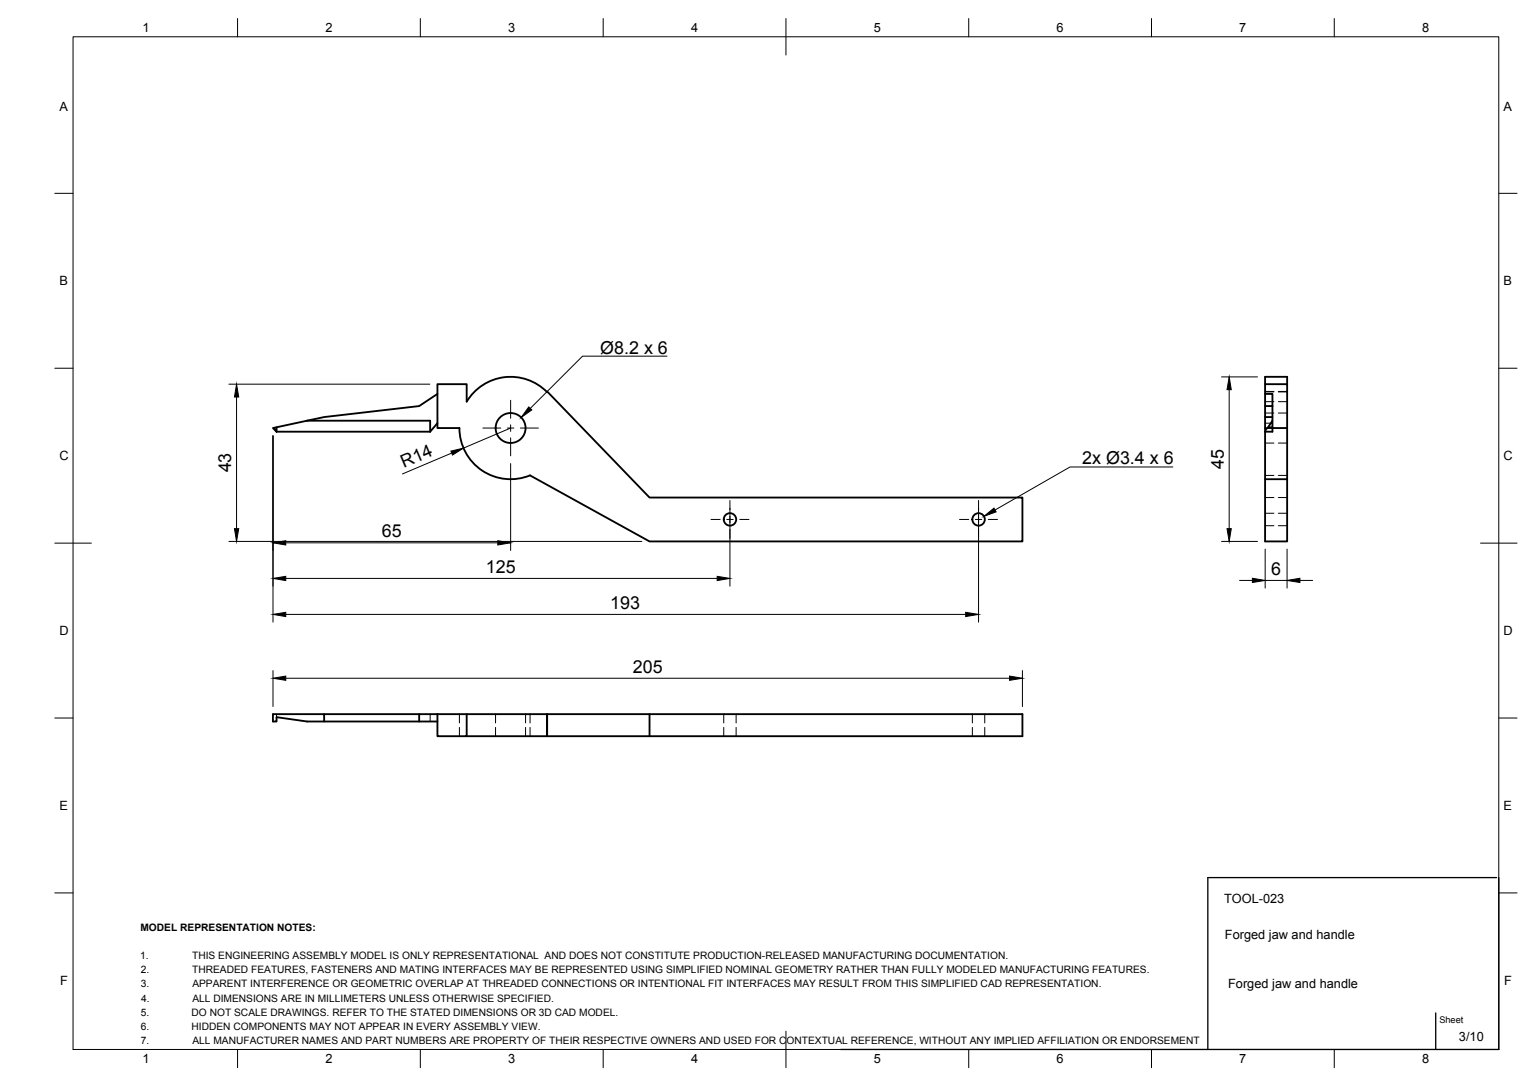
ISO-10303-21;
HEADER;
/* Generated by software containing ST-Developer
 * from STEP Tools, Inc. (www.steptools.com) 
 */

FILE_DESCRIPTION(
/* description */ (''),
/* implementation_level */ '2;1');

FILE_NAME(
/* name */ 'Forged jaw and handle.step',
/* time_stamp */ '2026-11-10T05:40:20-08:00',
/* author */ (''),
/* organization */ (''),
/* preprocessor_version */ 'ST-DEVELOPER v20.2',
/* originating_system */ 'Autodesk Translation Framework v15.17.0.0',
/* authorisation */ '');

FILE_SCHEMA (('AUTOMOTIVE_DESIGN { 1 0 10303 214 3 1 1 }'));
ENDSEC;

DATA;
#10=MECHANICAL_DESIGN_GEOMETRIC_PRESENTATION_REPRESENTATION('',(#572),#18580);
#554=SHAPE_REPRESENTATION_RELATIONSHIP('SRR','None',#18624,#563);
#563=ADVANCED_BREP_SHAPE_REPRESENTATION('',(#581),#18570);
#572=STYLED_ITEM('',(#18683),#581);
#581=MANIFOLD_SOLID_BREP('Body1',#6544);
#590=FACE_BOUND('',#1186,.T.);
#591=FACE_BOUND('',#1187,.T.);
#592=FACE_BOUND('',#1188,.T.);
#593=FACE_BOUND('',#1196,.T.);
#594=FACE_BOUND('',#1197,.T.);
#595=FACE_BOUND('',#1198,.T.);
#651=PLANE('',#6664);
#652=PLANE('',#6665);
#653=PLANE('',#6666);
#654=PLANE('',#6667);
#655=PLANE('',#6668);
#656=PLANE('',#6669);
#657=PLANE('',#6670);
#658=PLANE('',#6671);
#659=PLANE('',#6672);
#660=PLANE('',#6673);
#661=PLANE('',#6674);
#662=PLANE('',#6677);
#663=PLANE('',#6678);
#664=PLANE('',#6679);
#665=PLANE('',#6680);
#666=PLANE('',#6685);
#667=PLANE('',#6686);
#668=PLANE('',#6687);
#669=PLANE('',#6688);
#670=PLANE('',#6689);
#671=PLANE('',#6690);
#672=PLANE('',#6691);
#796=FACE_OUTER_BOUND('',#1172,.T.);
#797=FACE_OUTER_BOUND('',#1173,.T.);
#798=FACE_OUTER_BOUND('',#1174,.T.);
#799=FACE_OUTER_BOUND('',#1175,.T.);
#800=FACE_OUTER_BOUND('',#1176,.T.);
#801=FACE_OUTER_BOUND('',#1177,.T.);
#802=FACE_OUTER_BOUND('',#1178,.T.);
#803=FACE_OUTER_BOUND('',#1179,.T.);
#804=FACE_OUTER_BOUND('',#1180,.T.);
#805=FACE_OUTER_BOUND('',#1181,.T.);
#806=FACE_OUTER_BOUND('',#1182,.T.);
#807=FACE_OUTER_BOUND('',#1183,.T.);
#808=FACE_OUTER_BOUND('',#1184,.T.);
#809=FACE_OUTER_BOUND('',#1185,.T.);
#810=FACE_OUTER_BOUND('',#1189,.T.);
#811=FACE_OUTER_BOUND('',#1190,.T.);
#812=FACE_OUTER_BOUND('',#1191,.T.);
#813=FACE_OUTER_BOUND('',#1192,.T.);
#814=FACE_OUTER_BOUND('',#1193,.T.);
#815=FACE_OUTER_BOUND('',#1194,.T.);
#816=FACE_OUTER_BOUND('',#1195,.T.);
#817=FACE_OUTER_BOUND('',#1199,.T.);
#818=FACE_OUTER_BOUND('',#1200,.T.);
#819=FACE_OUTER_BOUND('',#1201,.T.);
#820=FACE_OUTER_BOUND('',#1202,.T.);
#821=FACE_OUTER_BOUND('',#1203,.T.);
#822=FACE_OUTER_BOUND('',#1204,.T.);
#1172=EDGE_LOOP('',(#4140,#4141,#4142,#4143));
#1173=EDGE_LOOP('',(#4144,#4145,#4146,#4147));
#1174=EDGE_LOOP('',(#4148,#4149,#4150,#4151));
#1175=EDGE_LOOP('',(#4152,#4153,#4154));
#1176=EDGE_LOOP('',(#4155,#4156,#4157,#4158,#4159));
#1177=EDGE_LOOP('',(#4160,#4161,#4162,#4163));
#1178=EDGE_LOOP('',(#4164,#4165,#4166));
#1179=EDGE_LOOP('',(#4167,#4168,#4169,#4170,#4171,#4172,#4173));
#1180=EDGE_LOOP('',(#4174,#4175,#4176,#4177));
#1181=EDGE_LOOP('',(#4178,#4179,#4180,#4181));
#1182=EDGE_LOOP('',(#4182,#4183,#4184,#4185));
#1183=EDGE_LOOP('',(#4186,#4187,#4188,#4189,#4190,#4191,#4192));
#1184=EDGE_LOOP('',(#4193,#4194,#4195,#4196));
#1185=EDGE_LOOP('',(#4197,#4198,#4199,#4200,#4201,#4202,#4203,#4204,#4205,
#4206,#4207,#4208,#4209,#4210,#4211,#4212,#4213,#4214,#4215));
#1186=EDGE_LOOP('',(#4216));
#1187=EDGE_LOOP('',(#4217));
#1188=EDGE_LOOP('',(#4218));
#1189=EDGE_LOOP('',(#4219,#4220,#4221,#4222));
#1190=EDGE_LOOP('',(#4223,#4224,#4225,#4226,#4227,#4228,#4229,#4230));
#1191=EDGE_LOOP('',(#4231,#4232,#4233,#4234));
#1192=EDGE_LOOP('',(#4235,#4236,#4237,#4238));
#1193=EDGE_LOOP('',(#4239,#4240,#4241,#4242));
#1194=EDGE_LOOP('',(#4243,#4244,#4245,#4246));
#1195=EDGE_LOOP('',(#4247,#4248,#4249,#4250,#4251,#4252,#4253,#4254,#4255,
#4256,#4257,#4258));
#1196=EDGE_LOOP('',(#4259));
#1197=EDGE_LOOP('',(#4260));
#1198=EDGE_LOOP('',(#4261));
#1199=EDGE_LOOP('',(#4262,#4263,#4264,#4265));
#1200=EDGE_LOOP('',(#4266,#4267,#4268,#4269));
#1201=EDGE_LOOP('',(#4270,#4271,#4272,#4273));
#1202=EDGE_LOOP('',(#4274,#4275,#4276,#4277));
#1203=EDGE_LOOP('',(#4278,#4279,#4280,#4281));
#1204=EDGE_LOOP('',(#4282,#4283,#4284,#4285));
#1609=LINE('',#8509,#2016);
#1610=LINE('',#8515,#2017);
#1611=LINE('',#8521,#2018);
#1612=LINE('',#8526,#2019);
#1613=LINE('',#8528,#2020);
#1614=LINE('',#8529,#2021);
#1615=LINE('',#8533,#2022);
#1616=LINE('',#8535,#2023);
#1617=LINE('',#8536,#2024);
#1618=LINE('',#8537,#2025);
#1619=LINE('',#8540,#2026);
#1620=LINE('',#8542,#2027);
#1621=LINE('',#8543,#2028);
#1622=LINE('',#8546,#2029);
#1623=LINE('',#8547,#2030);
#1624=LINE('',#8550,#2031);
#1625=LINE('',#8552,#2032);
#1626=LINE('',#8554,#2033);
#1627=LINE('',#8556,#2034);
#1628=LINE('',#8557,#2035);
#1629=LINE('',#8560,#2036);
#1630=LINE('',#8562,#2037);
#1631=LINE('',#8563,#2038);
#1632=LINE('',#8566,#2039);
#1633=LINE('',#8567,#2040);
#1634=LINE('',#8570,#2041);
#1635=LINE('',#8571,#2042);
#1636=LINE('',#8574,#2043);
#1637=LINE('',#8575,#2044);
#1638=LINE('',#8577,#2045);
#1639=LINE('',#8580,#2046);
#1640=LINE('',#8582,#2047);
#1641=LINE('',#8584,#2048);
#1642=LINE('',#8588,#2049);
#1643=LINE('',#8590,#2050);
#1644=LINE('',#8592,#2051);
#1645=LINE('',#8594,#2052);
#1646=LINE('',#8596,#2053);
#1647=LINE('',#8598,#2054);
#1648=LINE('',#8602,#2055);
#1649=LINE('',#8603,#2056);
#1650=LINE('',#8606,#2057);
#1651=LINE('',#8608,#2058);
#1652=LINE('',#8609,#2059);
#1653=LINE('',#8612,#2060);
#1654=LINE('',#8613,#2061);
#1655=LINE('',#8616,#2062);
#1656=LINE('',#8617,#2063);
#1657=LINE('',#8620,#2064);
#1658=LINE('',#8621,#2065);
#1659=LINE('',#8624,#2066);
#1660=LINE('',#8629,#2067);
#1661=LINE('',#8632,#2068);
#1662=LINE('',#8634,#2069);
#1663=LINE('',#8636,#2070);
#1664=LINE('',#8638,#2071);
#1665=LINE('',#8640,#2072);
#1666=LINE('',#8641,#2073);
#1667=LINE('',#8643,#2074);
#1668=LINE('',#8645,#2075);
#1669=LINE('',#8647,#2076);
#1670=LINE('',#8649,#2077);
#1671=LINE('',#8651,#2078);
#2016=VECTOR('',#7142,0.17);
#2017=VECTOR('',#7149,0.17);
#2018=VECTOR('',#7156,0.41);
#2019=VECTOR('',#7161,1.);
#2020=VECTOR('',#7162,1.);
#2021=VECTOR('',#7163,1.);
#2022=VECTOR('',#7166,1.);
#2023=VECTOR('',#7167,1.);
#2024=VECTOR('',#7168,1.);
#2025=VECTOR('',#7169,1.);
#2026=VECTOR('',#7172,1.);
#2027=VECTOR('',#7173,1.);
#2028=VECTOR('',#7174,1.);
#2029=VECTOR('',#7177,1.);
#2030=VECTOR('',#7178,1.);
#2031=VECTOR('',#7181,1.);
#2032=VECTOR('',#7182,1.);
#2033=VECTOR('',#7183,1.);
#2034=VECTOR('',#7184,1.);
#2035=VECTOR('',#7185,1.);
#2036=VECTOR('',#7188,1.);
#2037=VECTOR('',#7189,1.);
#2038=VECTOR('',#7190,1.);
#2039=VECTOR('',#7193,1.);
#2040=VECTOR('',#7194,1.);
#2041=VECTOR('',#7197,1.);
#2042=VECTOR('',#7198,1.);
#2043=VECTOR('',#7201,1.);
#2044=VECTOR('',#7202,1.);
#2045=VECTOR('',#7205,1.);
#2046=VECTOR('',#7208,1.);
#2047=VECTOR('',#7209,1.);
#2048=VECTOR('',#7210,1.);
#2049=VECTOR('',#7213,1.);
#2050=VECTOR('',#7214,1.);
#2051=VECTOR('',#7215,1.);
#2052=VECTOR('',#7216,1.);
#2053=VECTOR('',#7217,1.);
#2054=VECTOR('',#7218,1.);
#2055=VECTOR('',#7221,1.);
#2056=VECTOR('',#7222,1.);
#2057=VECTOR('',#7225,1.);
#2058=VECTOR('',#7226,1.);
#2059=VECTOR('',#7227,1.);
#2060=VECTOR('',#7230,1.);
#2061=VECTOR('',#7231,1.);
#2062=VECTOR('',#7234,1.);
#2063=VECTOR('',#7235,1.);
#2064=VECTOR('',#7238,1.);
#2065=VECTOR('',#7239,1.);
#2066=VECTOR('',#7242,1.);
#2067=VECTOR('',#7249,1.);
#2068=VECTOR('',#7252,1.);
#2069=VECTOR('',#7253,1.);
#2070=VECTOR('',#7254,1.);
#2071=VECTOR('',#7255,1.);
#2072=VECTOR('',#7256,1.);
#2073=VECTOR('',#7257,1.);
#2074=VECTOR('',#7260,1.);
#2075=VECTOR('',#7263,1.);
#2076=VECTOR('',#7266,1.);
#2077=VECTOR('',#7269,1.);
#2078=VECTOR('',#7272,1.);
#2423=CIRCLE('',#6656,0.17);
#2424=CIRCLE('',#6657,0.17);
#2425=CIRCLE('',#6659,0.17);
#2426=CIRCLE('',#6660,0.17);
#2427=CIRCLE('',#6662,0.41);
#2428=CIRCLE('',#6663,0.41);
#2429=CIRCLE('',#6675,1.4);
#2430=CIRCLE('',#6676,1.4);
#2431=CIRCLE('',#6682,1.4);
#2432=CIRCLE('',#6684,1.4);
#2581=VERTEX_POINT('',#8506);
#2582=VERTEX_POINT('',#8508);
#2583=VERTEX_POINT('',#8512);
#2584=VERTEX_POINT('',#8514);
#2585=VERTEX_POINT('',#8518);
#2586=VERTEX_POINT('',#8520);
#2587=VERTEX_POINT('',#8524);
#2588=VERTEX_POINT('',#8525);
#2589=VERTEX_POINT('',#8527);
#2590=VERTEX_POINT('',#8531);
#2591=VERTEX_POINT('',#8532);
#2592=VERTEX_POINT('',#8534);
#2593=VERTEX_POINT('',#8539);
#2594=VERTEX_POINT('',#8541);
#2595=VERTEX_POINT('',#8545);
#2596=VERTEX_POINT('',#8549);
#2597=VERTEX_POINT('',#8551);
#2598=VERTEX_POINT('',#8553);
#2599=VERTEX_POINT('',#8555);
#2600=VERTEX_POINT('',#8559);
#2601=VERTEX_POINT('',#8561);
#2602=VERTEX_POINT('',#8565);
#2603=VERTEX_POINT('',#8569);
#2604=VERTEX_POINT('',#8573);
#2605=VERTEX_POINT('',#8579);
#2606=VERTEX_POINT('',#8581);
#2607=VERTEX_POINT('',#8583);
#2608=VERTEX_POINT('',#8585);
#2609=VERTEX_POINT('',#8587);
#2610=VERTEX_POINT('',#8589);
#2611=VERTEX_POINT('',#8591);
#2612=VERTEX_POINT('',#8593);
#2613=VERTEX_POINT('',#8595);
#2614=VERTEX_POINT('',#8597);
#2615=VERTEX_POINT('',#8599);
#2616=VERTEX_POINT('',#8601);
#2617=VERTEX_POINT('',#8605);
#2618=VERTEX_POINT('',#8607);
#2619=VERTEX_POINT('',#8611);
#2620=VERTEX_POINT('',#8615);
#2621=VERTEX_POINT('',#8619);
#2622=VERTEX_POINT('',#8623);
#2623=VERTEX_POINT('',#8627);
#2624=VERTEX_POINT('',#8631);
#2625=VERTEX_POINT('',#8633);
#2626=VERTEX_POINT('',#8635);
#2627=VERTEX_POINT('',#8637);
#2628=VERTEX_POINT('',#8639);
#3193=EDGE_CURVE('',#2581,#2581,#2423,.T.);
#3194=EDGE_CURVE('',#2581,#2582,#1609,.T.);
#3195=EDGE_CURVE('',#2582,#2582,#2424,.T.);
#3196=EDGE_CURVE('',#2583,#2583,#2425,.T.);
#3197=EDGE_CURVE('',#2583,#2584,#1610,.T.);
#3198=EDGE_CURVE('',#2584,#2584,#2426,.T.);
#3199=EDGE_CURVE('',#2585,#2585,#2427,.T.);
#3200=EDGE_CURVE('',#2585,#2586,#1611,.T.);
#3201=EDGE_CURVE('',#2586,#2586,#2428,.T.);
#3202=EDGE_CURVE('',#2587,#2588,#1612,.T.);
#3203=EDGE_CURVE('',#2589,#2587,#1613,.T.);
#3204=EDGE_CURVE('',#2589,#2588,#1614,.T.);
#3205=EDGE_CURVE('',#2590,#2591,#1615,.T.);
#3206=EDGE_CURVE('',#2592,#2590,#1616,.T.);
#3207=EDGE_CURVE('',#2589,#2592,#1617,.T.);
#3208=EDGE_CURVE('',#2591,#2587,#1618,.T.);
#3209=EDGE_CURVE('',#2593,#2590,#1619,.T.);
#3210=EDGE_CURVE('',#2594,#2593,#1620,.T.);
#3211=EDGE_CURVE('',#2592,#2594,#1621,.T.);
#3212=EDGE_CURVE('',#2593,#2595,#1622,.T.);
#3213=EDGE_CURVE('',#2595,#2594,#1623,.T.);
#3214=EDGE_CURVE('',#2588,#2596,#1624,.T.);
#3215=EDGE_CURVE('',#2597,#2596,#1625,.T.);
#3216=EDGE_CURVE('',#2597,#2598,#1626,.T.);
#3217=EDGE_CURVE('',#2598,#2599,#1627,.T.);
#3218=EDGE_CURVE('',#2599,#2591,#1628,.T.);
#3219=EDGE_CURVE('',#2600,#2597,#1629,.T.);
#3220=EDGE_CURVE('',#2601,#2600,#1630,.T.);
#3221=EDGE_CURVE('',#2601,#2598,#1631,.T.);
#3222=EDGE_CURVE('',#2596,#2602,#1632,.T.);
#3223=EDGE_CURVE('',#2602,#2589,#1633,.T.);
#3224=EDGE_CURVE('',#2592,#2603,#1634,.T.);
#3225=EDGE_CURVE('',#2603,#2595,#1635,.T.);
#3226=EDGE_CURVE('',#2604,#2599,#1636,.T.);
#3227=EDGE_CURVE('',#2603,#2604,#1637,.T.);
#3228=EDGE_CURVE('',#2604,#2601,#1638,.T.);
#3229=EDGE_CURVE('',#2600,#2605,#1639,.T.);
#3230=EDGE_CURVE('',#2605,#2606,#1640,.T.);
#3231=EDGE_CURVE('',#2606,#2607,#1641,.T.);
#3232=EDGE_CURVE('',#2608,#2607,#2429,.T.);
#3233=EDGE_CURVE('',#2609,#2608,#1642,.T.);
#3234=EDGE_CURVE('',#2610,#2609,#1643,.T.);
#3235=EDGE_CURVE('',#2611,#2610,#1644,.T.);
#3236=EDGE_CURVE('',#2612,#2611,#1645,.T.);
#3237=EDGE_CURVE('',#2613,#2612,#1646,.T.);
#3238=EDGE_CURVE('',#2614,#2613,#1647,.T.);
#3239=EDGE_CURVE('',#2615,#2614,#2430,.T.);
#3240=EDGE_CURVE('',#2615,#2616,#1648,.T.);
#3241=EDGE_CURVE('',#2616,#2602,#1649,.T.);
#3242=EDGE_CURVE('',#2617,#2615,#1650,.T.);
#3243=EDGE_CURVE('',#2618,#2617,#1651,.T.);
#3244=EDGE_CURVE('',#2616,#2618,#1652,.T.);
#3245=EDGE_CURVE('',#2619,#2618,#1653,.T.);
#3246=EDGE_CURVE('',#2605,#2619,#1654,.T.);
#3247=EDGE_CURVE('',#2620,#2619,#1655,.T.);
#3248=EDGE_CURVE('',#2606,#2620,#1656,.T.);
#3249=EDGE_CURVE('',#2607,#2621,#1657,.T.);
#3250=EDGE_CURVE('',#2621,#2620,#1658,.T.);
#3251=EDGE_CURVE('',#2614,#2622,#1659,.T.);
#3252=EDGE_CURVE('',#2617,#2622,#2431,.T.);
#3253=EDGE_CURVE('',#2623,#2621,#2432,.T.);
#3254=EDGE_CURVE('',#2623,#2608,#1660,.T.);
#3255=EDGE_CURVE('',#2622,#2624,#1661,.T.);
#3256=EDGE_CURVE('',#2624,#2625,#1662,.T.);
#3257=EDGE_CURVE('',#2625,#2626,#1663,.T.);
#3258=EDGE_CURVE('',#2626,#2627,#1664,.T.);
#3259=EDGE_CURVE('',#2627,#2628,#1665,.T.);
#3260=EDGE_CURVE('',#2628,#2623,#1666,.T.);
#3261=EDGE_CURVE('',#2613,#2624,#1667,.T.);
#3262=EDGE_CURVE('',#2609,#2628,#1668,.T.);
#3263=EDGE_CURVE('',#2610,#2627,#1669,.T.);
#3264=EDGE_CURVE('',#2611,#2626,#1670,.T.);
#3265=EDGE_CURVE('',#2612,#2625,#1671,.T.);
#4140=ORIENTED_EDGE('',*,*,#3193,.F.);
#4141=ORIENTED_EDGE('',*,*,#3194,.T.);
#4142=ORIENTED_EDGE('',*,*,#3195,.F.);
#4143=ORIENTED_EDGE('',*,*,#3194,.F.);
#4144=ORIENTED_EDGE('',*,*,#3196,.F.);
#4145=ORIENTED_EDGE('',*,*,#3197,.T.);
#4146=ORIENTED_EDGE('',*,*,#3198,.F.);
#4147=ORIENTED_EDGE('',*,*,#3197,.F.);
#4148=ORIENTED_EDGE('',*,*,#3199,.F.);
#4149=ORIENTED_EDGE('',*,*,#3200,.T.);
#4150=ORIENTED_EDGE('',*,*,#3201,.F.);
#4151=ORIENTED_EDGE('',*,*,#3200,.F.);
#4152=ORIENTED_EDGE('',*,*,#3202,.F.);
#4153=ORIENTED_EDGE('',*,*,#3203,.F.);
#4154=ORIENTED_EDGE('',*,*,#3204,.T.);
#4155=ORIENTED_EDGE('',*,*,#3205,.F.);
#4156=ORIENTED_EDGE('',*,*,#3206,.F.);
#4157=ORIENTED_EDGE('',*,*,#3207,.F.);
#4158=ORIENTED_EDGE('',*,*,#3203,.T.);
#4159=ORIENTED_EDGE('',*,*,#3208,.F.);
#4160=ORIENTED_EDGE('',*,*,#3209,.F.);
#4161=ORIENTED_EDGE('',*,*,#3210,.F.);
#4162=ORIENTED_EDGE('',*,*,#3211,.F.);
#4163=ORIENTED_EDGE('',*,*,#3206,.T.);
#4164=ORIENTED_EDGE('',*,*,#3210,.T.);
#4165=ORIENTED_EDGE('',*,*,#3212,.T.);
#4166=ORIENTED_EDGE('',*,*,#3213,.T.);
#4167=ORIENTED_EDGE('',*,*,#3202,.T.);
#4168=ORIENTED_EDGE('',*,*,#3214,.T.);
#4169=ORIENTED_EDGE('',*,*,#3215,.F.);
#4170=ORIENTED_EDGE('',*,*,#3216,.T.);
#4171=ORIENTED_EDGE('',*,*,#3217,.T.);
#4172=ORIENTED_EDGE('',*,*,#3218,.T.);
#4173=ORIENTED_EDGE('',*,*,#3208,.T.);
#4174=ORIENTED_EDGE('',*,*,#3219,.F.);
#4175=ORIENTED_EDGE('',*,*,#3220,.F.);
#4176=ORIENTED_EDGE('',*,*,#3221,.T.);
#4177=ORIENTED_EDGE('',*,*,#3216,.F.);
#4178=ORIENTED_EDGE('',*,*,#3222,.F.);
#4179=ORIENTED_EDGE('',*,*,#3214,.F.);
#4180=ORIENTED_EDGE('',*,*,#3204,.F.);
#4181=ORIENTED_EDGE('',*,*,#3223,.F.);
#4182=ORIENTED_EDGE('',*,*,#3224,.F.);
#4183=ORIENTED_EDGE('',*,*,#3211,.T.);
#4184=ORIENTED_EDGE('',*,*,#3213,.F.);
#4185=ORIENTED_EDGE('',*,*,#3225,.F.);
#4186=ORIENTED_EDGE('',*,*,#3205,.T.);
#4187=ORIENTED_EDGE('',*,*,#3218,.F.);
#4188=ORIENTED_EDGE('',*,*,#3226,.F.);
#4189=ORIENTED_EDGE('',*,*,#3227,.F.);
#4190=ORIENTED_EDGE('',*,*,#3225,.T.);
#4191=ORIENTED_EDGE('',*,*,#3212,.F.);
#4192=ORIENTED_EDGE('',*,*,#3209,.T.);
#4193=ORIENTED_EDGE('',*,*,#3228,.F.);
#4194=ORIENTED_EDGE('',*,*,#3226,.T.);
#4195=ORIENTED_EDGE('',*,*,#3217,.F.);
#4196=ORIENTED_EDGE('',*,*,#3221,.F.);
#4197=ORIENTED_EDGE('',*,*,#3229,.T.);
#4198=ORIENTED_EDGE('',*,*,#3230,.T.);
#4199=ORIENTED_EDGE('',*,*,#3231,.T.);
#4200=ORIENTED_EDGE('',*,*,#3232,.F.);
#4201=ORIENTED_EDGE('',*,*,#3233,.F.);
#4202=ORIENTED_EDGE('',*,*,#3234,.F.);
#4203=ORIENTED_EDGE('',*,*,#3235,.F.);
#4204=ORIENTED_EDGE('',*,*,#3236,.F.);
#4205=ORIENTED_EDGE('',*,*,#3237,.F.);
#4206=ORIENTED_EDGE('',*,*,#3238,.F.);
#4207=ORIENTED_EDGE('',*,*,#3239,.F.);
#4208=ORIENTED_EDGE('',*,*,#3240,.T.);
#4209=ORIENTED_EDGE('',*,*,#3241,.T.);
#4210=ORIENTED_EDGE('',*,*,#3223,.T.);
#4211=ORIENTED_EDGE('',*,*,#3207,.T.);
#4212=ORIENTED_EDGE('',*,*,#3224,.T.);
#4213=ORIENTED_EDGE('',*,*,#3227,.T.);
#4214=ORIENTED_EDGE('',*,*,#3228,.T.);
#4215=ORIENTED_EDGE('',*,*,#3220,.T.);
#4216=ORIENTED_EDGE('',*,*,#3195,.T.);
#4217=ORIENTED_EDGE('',*,*,#3198,.T.);
#4218=ORIENTED_EDGE('',*,*,#3201,.T.);
#4219=ORIENTED_EDGE('',*,*,#3242,.F.);
#4220=ORIENTED_EDGE('',*,*,#3243,.F.);
#4221=ORIENTED_EDGE('',*,*,#3244,.F.);
#4222=ORIENTED_EDGE('',*,*,#3240,.F.);
#4223=ORIENTED_EDGE('',*,*,#3222,.T.);
#4224=ORIENTED_EDGE('',*,*,#3241,.F.);
#4225=ORIENTED_EDGE('',*,*,#3244,.T.);
#4226=ORIENTED_EDGE('',*,*,#3245,.F.);
#4227=ORIENTED_EDGE('',*,*,#3246,.F.);
#4228=ORIENTED_EDGE('',*,*,#3229,.F.);
#4229=ORIENTED_EDGE('',*,*,#3219,.T.);
#4230=ORIENTED_EDGE('',*,*,#3215,.T.);
#4231=ORIENTED_EDGE('',*,*,#3230,.F.);
#4232=ORIENTED_EDGE('',*,*,#3246,.T.);
#4233=ORIENTED_EDGE('',*,*,#3247,.F.);
#4234=ORIENTED_EDGE('',*,*,#3248,.F.);
#4235=ORIENTED_EDGE('',*,*,#3249,.F.);
#4236=ORIENTED_EDGE('',*,*,#3231,.F.);
#4237=ORIENTED_EDGE('',*,*,#3248,.T.);
#4238=ORIENTED_EDGE('',*,*,#3250,.F.);
#4239=ORIENTED_EDGE('',*,*,#3242,.T.);
#4240=ORIENTED_EDGE('',*,*,#3239,.T.);
#4241=ORIENTED_EDGE('',*,*,#3251,.T.);
#4242=ORIENTED_EDGE('',*,*,#3252,.F.);
#4243=ORIENTED_EDGE('',*,*,#3249,.T.);
#4244=ORIENTED_EDGE('',*,*,#3253,.F.);
#4245=ORIENTED_EDGE('',*,*,#3254,.T.);
#4246=ORIENTED_EDGE('',*,*,#3232,.T.);
#4247=ORIENTED_EDGE('',*,*,#3252,.T.);
#4248=ORIENTED_EDGE('',*,*,#3255,.T.);
#4249=ORIENTED_EDGE('',*,*,#3256,.T.);
#4250=ORIENTED_EDGE('',*,*,#3257,.T.);
#4251=ORIENTED_EDGE('',*,*,#3258,.T.);
#4252=ORIENTED_EDGE('',*,*,#3259,.T.);
#4253=ORIENTED_EDGE('',*,*,#3260,.T.);
#4254=ORIENTED_EDGE('',*,*,#3253,.T.);
#4255=ORIENTED_EDGE('',*,*,#3250,.T.);
#4256=ORIENTED_EDGE('',*,*,#3247,.T.);
#4257=ORIENTED_EDGE('',*,*,#3245,.T.);
#4258=ORIENTED_EDGE('',*,*,#3243,.T.);
#4259=ORIENTED_EDGE('',*,*,#3193,.T.);
#4260=ORIENTED_EDGE('',*,*,#3196,.T.);
#4261=ORIENTED_EDGE('',*,*,#3199,.T.);
#4262=ORIENTED_EDGE('',*,*,#3251,.F.);
#4263=ORIENTED_EDGE('',*,*,#3238,.T.);
#4264=ORIENTED_EDGE('',*,*,#3261,.T.);
#4265=ORIENTED_EDGE('',*,*,#3255,.F.);
#4266=ORIENTED_EDGE('',*,*,#3254,.F.);
#4267=ORIENTED_EDGE('',*,*,#3260,.F.);
#4268=ORIENTED_EDGE('',*,*,#3262,.F.);
#4269=ORIENTED_EDGE('',*,*,#3233,.T.);
#4270=ORIENTED_EDGE('',*,*,#3234,.T.);
#4271=ORIENTED_EDGE('',*,*,#3262,.T.);
#4272=ORIENTED_EDGE('',*,*,#3259,.F.);
#4273=ORIENTED_EDGE('',*,*,#3263,.F.);
#4274=ORIENTED_EDGE('',*,*,#3235,.T.);
#4275=ORIENTED_EDGE('',*,*,#3263,.T.);
#4276=ORIENTED_EDGE('',*,*,#3258,.F.);
#4277=ORIENTED_EDGE('',*,*,#3264,.F.);
#4278=ORIENTED_EDGE('',*,*,#3236,.T.);
#4279=ORIENTED_EDGE('',*,*,#3264,.T.);
#4280=ORIENTED_EDGE('',*,*,#3257,.F.);
#4281=ORIENTED_EDGE('',*,*,#3265,.F.);
#4282=ORIENTED_EDGE('',*,*,#3237,.T.);
#4283=ORIENTED_EDGE('',*,*,#3265,.T.);
#4284=ORIENTED_EDGE('',*,*,#3256,.F.);
#4285=ORIENTED_EDGE('',*,*,#3261,.F.);
#6034=CYLINDRICAL_SURFACE('',#6655,0.17);
#6035=CYLINDRICAL_SURFACE('',#6658,0.17);
#6036=CYLINDRICAL_SURFACE('',#6661,0.41);
#6037=CYLINDRICAL_SURFACE('',#6681,1.4);
#6038=CYLINDRICAL_SURFACE('',#6683,1.4);
#6168=ADVANCED_FACE('',(#796),#6034,.F.);
#6169=ADVANCED_FACE('',(#797),#6035,.F.);
#6170=ADVANCED_FACE('',(#798),#6036,.F.);
#6171=ADVANCED_FACE('',(#799),#651,.F.);
#6172=ADVANCED_FACE('',(#800),#652,.F.);
#6173=ADVANCED_FACE('',(#801),#653,.T.);
#6174=ADVANCED_FACE('',(#802),#654,.T.);
#6175=ADVANCED_FACE('',(#803),#655,.T.);
#6176=ADVANCED_FACE('',(#804),#656,.T.);
#6177=ADVANCED_FACE('',(#805),#657,.T.);
#6178=ADVANCED_FACE('',(#806),#658,.T.);
#6179=ADVANCED_FACE('',(#807),#659,.T.);
#6180=ADVANCED_FACE('',(#808),#660,.T.);
#6181=ADVANCED_FACE('',(#809,#590,#591,#592),#661,.F.);
#6182=ADVANCED_FACE('',(#810),#662,.T.);
#6183=ADVANCED_FACE('',(#811),#663,.T.);
#6184=ADVANCED_FACE('',(#812),#664,.T.);
#6185=ADVANCED_FACE('',(#813),#665,.T.);
#6186=ADVANCED_FACE('',(#814),#6037,.T.);
#6187=ADVANCED_FACE('',(#815),#6038,.T.);
#6188=ADVANCED_FACE('',(#816,#593,#594,#595),#666,.T.);
#6189=ADVANCED_FACE('',(#817),#667,.T.);
#6190=ADVANCED_FACE('',(#818),#668,.T.);
#6191=ADVANCED_FACE('',(#819),#669,.T.);
#6192=ADVANCED_FACE('',(#820),#670,.T.);
#6193=ADVANCED_FACE('',(#821),#671,.T.);
#6194=ADVANCED_FACE('',(#822),#672,.T.);
#6544=CLOSED_SHELL('',(#6168,#6169,#6170,#6171,#6172,#6173,#6174,#6175,
#6176,#6177,#6178,#6179,#6180,#6181,#6182,#6183,#6184,#6185,#6186,#6187,
#6188,#6189,#6190,#6191,#6192,#6193,#6194));
#6654=AXIS2_PLACEMENT_3D('',#8504,#7136,#7137);
#6655=AXIS2_PLACEMENT_3D('',#8505,#7138,#7139);
#6656=AXIS2_PLACEMENT_3D('',#8507,#7140,#7141);
#6657=AXIS2_PLACEMENT_3D('',#8510,#7143,#7144);
#6658=AXIS2_PLACEMENT_3D('',#8511,#7145,#7146);
#6659=AXIS2_PLACEMENT_3D('',#8513,#7147,#7148);
#6660=AXIS2_PLACEMENT_3D('',#8516,#7150,#7151);
#6661=AXIS2_PLACEMENT_3D('',#8517,#7152,#7153);
#6662=AXIS2_PLACEMENT_3D('',#8519,#7154,#7155);
#6663=AXIS2_PLACEMENT_3D('',#8522,#7157,#7158);
#6664=AXIS2_PLACEMENT_3D('',#8523,#7159,#7160);
#6665=AXIS2_PLACEMENT_3D('',#8530,#7164,#7165);
#6666=AXIS2_PLACEMENT_3D('',#8538,#7170,#7171);
#6667=AXIS2_PLACEMENT_3D('',#8544,#7175,#7176);
#6668=AXIS2_PLACEMENT_3D('',#8548,#7179,#7180);
#6669=AXIS2_PLACEMENT_3D('',#8558,#7186,#7187);
#6670=AXIS2_PLACEMENT_3D('',#8564,#7191,#7192);
#6671=AXIS2_PLACEMENT_3D('',#8568,#7195,#7196);
#6672=AXIS2_PLACEMENT_3D('',#8572,#7199,#7200);
#6673=AXIS2_PLACEMENT_3D('',#8576,#7203,#7204);
#6674=AXIS2_PLACEMENT_3D('',#8578,#7206,#7207);
#6675=AXIS2_PLACEMENT_3D('',#8586,#7211,#7212);
#6676=AXIS2_PLACEMENT_3D('',#8600,#7219,#7220);
#6677=AXIS2_PLACEMENT_3D('',#8604,#7223,#7224);
#6678=AXIS2_PLACEMENT_3D('',#8610,#7228,#7229);
#6679=AXIS2_PLACEMENT_3D('',#8614,#7232,#7233);
#6680=AXIS2_PLACEMENT_3D('',#8618,#7236,#7237);
#6681=AXIS2_PLACEMENT_3D('',#8622,#7240,#7241);
#6682=AXIS2_PLACEMENT_3D('',#8625,#7243,#7244);
#6683=AXIS2_PLACEMENT_3D('',#8626,#7245,#7246);
#6684=AXIS2_PLACEMENT_3D('',#8628,#7247,#7248);
#6685=AXIS2_PLACEMENT_3D('',#8630,#7250,#7251);
#6686=AXIS2_PLACEMENT_3D('',#8642,#7258,#7259);
#6687=AXIS2_PLACEMENT_3D('',#8644,#7261,#7262);
#6688=AXIS2_PLACEMENT_3D('',#8646,#7264,#7265);
#6689=AXIS2_PLACEMENT_3D('',#8648,#7267,#7268);
#6690=AXIS2_PLACEMENT_3D('',#8650,#7270,#7271);
#6691=AXIS2_PLACEMENT_3D('',#8652,#7273,#7274);
#7136=DIRECTION('axis',(0.,0.,1.));
#7137=DIRECTION('refdir',(1.,0.,0.));
#7138=DIRECTION('center_axis',(0.,0.,-1.));
#7139=DIRECTION('ref_axis',(1.,0.,0.));
#7140=DIRECTION('center_axis',(0.,0.,-1.));
#7141=DIRECTION('ref_axis',(1.,0.,0.));
#7142=DIRECTION('',(0.,0.,-1.));
#7143=DIRECTION('center_axis',(0.,0.,1.));
#7144=DIRECTION('ref_axis',(1.,0.,0.));
#7145=DIRECTION('center_axis',(0.,0.,-1.));
#7146=DIRECTION('ref_axis',(1.,0.,0.));
#7147=DIRECTION('center_axis',(0.,0.,-1.));
#7148=DIRECTION('ref_axis',(1.,0.,0.));
#7149=DIRECTION('',(0.,0.,-1.));
#7150=DIRECTION('center_axis',(0.,0.,1.));
#7151=DIRECTION('ref_axis',(1.,0.,0.));
#7152=DIRECTION('center_axis',(0.,0.,-1.));
#7153=DIRECTION('ref_axis',(1.,0.,0.));
#7154=DIRECTION('center_axis',(0.,0.,-1.));
#7155=DIRECTION('ref_axis',(1.,0.,0.));
#7156=DIRECTION('',(0.,0.,-1.));
#7157=DIRECTION('center_axis',(0.,0.,1.));
#7158=DIRECTION('ref_axis',(1.,0.,0.));
#7159=DIRECTION('center_axis',(1.,0.,0.));
#7160=DIRECTION('ref_axis',(0.,0.,-1.));
#7161=DIRECTION('',(0.,-1.,0.));
#7162=DIRECTION('',(0.,0.832050294337844,0.554700196225229));
#7163=DIRECTION('',(0.,0.,1.));
#7164=DIRECTION('center_axis',(0.,0.554700196225229,-0.832050294337844));
#7165=DIRECTION('ref_axis',(0.,0.832050294337844,0.554700196225229));
#7166=DIRECTION('',(0.968400249412505,0.207514339159822,0.138342892773215));
#7167=DIRECTION('',(0.,0.832050294337844,0.554700196225229));
#7168=DIRECTION('',(-1.,0.,0.));
#7169=DIRECTION('',(1.,0.,0.));
#7170=DIRECTION('center_axis',(1.,0.,0.));
#7171=DIRECTION('ref_axis',(0.,2.22044604925031E-16,1.));
#7172=DIRECTION('',(0.,0.,-1.));
#7173=DIRECTION('',(0.,1.,0.));
#7174=DIRECTION('',(0.,0.,1.));
#7175=DIRECTION('center_axis',(0.,0.,1.));
#7176=DIRECTION('ref_axis',(1.,0.,0.));
#7177=DIRECTION('',(-0.97780241407741,-0.209529088730873,0.));
#7178=DIRECTION('',(0.707106781186546,-0.707106781186549,0.));
#7179=DIRECTION('center_axis',(0.,0.,1.));
#7180=DIRECTION('ref_axis',(1.,0.,0.));
#7181=DIRECTION('',(0.650791373455969,0.759256602365297,0.));
#7182=DIRECTION('',(0.,-1.,0.));
#7183=DIRECTION('',(-0.832050294337844,-0.554700196225229,0.));
#7184=DIRECTION('',(-0.993408935871131,-0.114624107985131,0.));
#7185=DIRECTION('',(-0.97780241407741,-0.209529088730873,0.));
#7186=DIRECTION('center_axis',(-0.554700196225229,0.832050294337844,0.));
#7187=DIRECTION('ref_axis',(-0.832050294337844,-0.554700196225229,0.));
#7188=DIRECTION('',(0.,0.,1.));
#7189=DIRECTION('',(0.832050294337844,0.554700196225229,0.));
#7190=DIRECTION('',(0.,0.,1.));
#7191=DIRECTION('center_axis',(0.759256602365297,-0.650791373455969,0.));
#7192=DIRECTION('ref_axis',(0.650791373455969,0.759256602365297,0.));
#7193=DIRECTION('',(0.,0.,-1.));
#7194=DIRECTION('',(-0.650791373455969,-0.759256602365297,0.));
#7195=DIRECTION('center_axis',(-0.707106781186549,-0.707106781186546,0.));
#7196=DIRECTION('ref_axis',(0.707106781186546,-0.707106781186549,0.));
#7197=DIRECTION('',(-0.707106781186546,0.707106781186549,0.));
#7198=DIRECTION('',(0.,0.,1.));
#7199=DIRECTION('center_axis',(-0.209529088730873,0.97780241407741,0.));
#7200=DIRECTION('ref_axis',(-0.97780241407741,-0.209529088730873,0.));
#7201=DIRECTION('',(0.,0.,1.));
#7202=DIRECTION('',(0.97780241407741,0.209529088730873,0.));
#7203=DIRECTION('center_axis',(-0.114624107985131,0.993408935871131,0.));
#7204=DIRECTION('ref_axis',(-0.993408935871131,-0.114624107985131,0.));
#7205=DIRECTION('',(0.993408935871131,0.114624107985131,0.));
#7206=DIRECTION('center_axis',(0.,0.,1.));
#7207=DIRECTION('ref_axis',(1.,0.,0.));
#7208=DIRECTION('',(0.,1.,0.));
#7209=DIRECTION('',(1.,0.,0.));
#7210=DIRECTION('',(0.,-1.,0.));
#7211=DIRECTION('center_axis',(0.,0.,1.));
#7212=DIRECTION('ref_axis',(1.,0.,0.));
#7213=DIRECTION('',(-0.447213595499958,-0.894427190999916,0.));
#7214=DIRECTION('',(-0.694594513699567,0.719401460617409,0.));
#7215=DIRECTION('',(-1.,0.,0.));
#7216=DIRECTION('',(0.,1.,0.));
#7217=DIRECTION('',(1.,0.,0.));
#7218=DIRECTION('',(0.87524153543927,-0.483686111690123,0.));
#7219=DIRECTION('center_axis',(0.,0.,1.));
#7220=DIRECTION('ref_axis',(1.,0.,0.));
#7221=DIRECTION('',(-1.,0.,0.));
#7222=DIRECTION('',(0.,1.,0.));
#7223=DIRECTION('center_axis',(0.,-1.,0.));
#7224=DIRECTION('ref_axis',(1.,0.,0.));
#7225=DIRECTION('',(0.,0.,-1.));
#7226=DIRECTION('',(1.,0.,0.));
#7227=DIRECTION('',(0.,0.,1.));
#7228=DIRECTION('center_axis',(-1.,0.,0.));
#7229=DIRECTION('ref_axis',(0.,-1.,0.));
#7230=DIRECTION('',(0.,-1.,0.));
#7231=DIRECTION('',(0.,0.,1.));
#7232=DIRECTION('center_axis',(0.,1.,0.));
#7233=DIRECTION('ref_axis',(-1.,0.,0.));
#7234=DIRECTION('',(-1.,0.,0.));
#7235=DIRECTION('',(0.,0.,1.));
#7236=DIRECTION('center_axis',(1.,0.,0.));
#7237=DIRECTION('ref_axis',(0.,1.,0.));
#7238=DIRECTION('',(0.,0.,1.));
#7239=DIRECTION('',(0.,1.,0.));
#7240=DIRECTION('center_axis',(0.,0.,1.));
#7241=DIRECTION('ref_axis',(1.,0.,0.));
#7242=DIRECTION('',(0.,0.,1.));
#7243=DIRECTION('center_axis',(0.,0.,1.));
#7244=DIRECTION('ref_axis',(1.,0.,0.));
#7245=DIRECTION('center_axis',(0.,0.,1.));
#7246=DIRECTION('ref_axis',(1.,0.,0.));
#7247=DIRECTION('center_axis',(0.,0.,1.));
#7248=DIRECTION('ref_axis',(1.,0.,0.));
#7249=DIRECTION('',(0.,0.,-1.));
#7250=DIRECTION('center_axis',(0.,0.,1.));
#7251=DIRECTION('ref_axis',(1.,0.,0.));
#7252=DIRECTION('',(0.87524153543927,-0.483686111690123,0.));
#7253=DIRECTION('',(1.,0.,0.));
#7254=DIRECTION('',(0.,1.,0.));
#7255=DIRECTION('',(-1.,0.,0.));
#7256=DIRECTION('',(-0.694594513699567,0.719401460617409,0.));
#7257=DIRECTION('',(-0.447213595499958,-0.894427190999916,0.));
#7258=DIRECTION('center_axis',(-0.483686111690123,-0.87524153543927,0.));
#7259=DIRECTION('ref_axis',(0.87524153543927,-0.483686111690123,0.));
#7260=DIRECTION('',(0.,0.,1.));
#7261=DIRECTION('center_axis',(-0.894427190999916,0.447213595499958,0.));
#7262=DIRECTION('ref_axis',(-0.447213595499958,-0.894427190999916,0.));
#7263=DIRECTION('',(0.,0.,1.));
#7264=DIRECTION('center_axis',(0.719401460617409,0.694594513699567,0.));
#7265=DIRECTION('ref_axis',(-0.694594513699567,0.719401460617409,0.));
#7266=DIRECTION('',(0.,0.,1.));
#7267=DIRECTION('center_axis',(0.,1.,0.));
#7268=DIRECTION('ref_axis',(-1.,0.,0.));
#7269=DIRECTION('',(0.,0.,1.));
#7270=DIRECTION('center_axis',(1.,0.,0.));
#7271=DIRECTION('ref_axis',(0.,1.,0.));
#7272=DIRECTION('',(0.,0.,1.));
#7273=DIRECTION('center_axis',(0.,-1.,0.));
#7274=DIRECTION('ref_axis',(1.,0.,0.));
#8504=CARTESIAN_POINT('',(0.,0.,0.));
#8505=CARTESIAN_POINT('Origin',(6.,-2.5,0.3));
#8506=CARTESIAN_POINT('',(5.83,-2.5,0.6));
#8507=CARTESIAN_POINT('Origin',(6.,-2.5,0.6));
#8508=CARTESIAN_POINT('',(5.83,-2.5,0.));
#8509=CARTESIAN_POINT('',(5.83,-2.5,0.3));
#8510=CARTESIAN_POINT('Origin',(6.,-2.5,0.));
#8511=CARTESIAN_POINT('Origin',(12.8,-2.5,0.3));
#8512=CARTESIAN_POINT('',(12.63,-2.5,0.6));
#8513=CARTESIAN_POINT('Origin',(12.8,-2.5,0.6));
#8514=CARTESIAN_POINT('',(12.63,-2.5,0.));
#8515=CARTESIAN_POINT('',(12.63,-2.5,0.3));
#8516=CARTESIAN_POINT('Origin',(12.8,-2.5,0.));
#8517=CARTESIAN_POINT('Origin',(0.,0.,0.3));
#8518=CARTESIAN_POINT('',(-0.41,5.02105187650415E-17,0.6));
#8519=CARTESIAN_POINT('Origin',(0.,0.,0.6));
#8520=CARTESIAN_POINT('',(-0.41,5.02105187650415E-17,0.));
#8521=CARTESIAN_POINT('',(-0.41,5.02105187650415E-17,0.3));
#8522=CARTESIAN_POINT('Origin',(0.,0.,0.));
#8523=CARTESIAN_POINT('Origin',(-2.2,0.025,0.125));
#8524=CARTESIAN_POINT('',(-2.2,0.2,0.2));
#8525=CARTESIAN_POINT('',(-2.2,-0.0999999999999999,0.2));
#8526=CARTESIAN_POINT('',(-2.2,0.2875,0.2));
#8527=CARTESIAN_POINT('',(-2.2,-0.1,0.));
#8528=CARTESIAN_POINT('',(-2.2,-0.1,0.));
#8529=CARTESIAN_POINT('',(-2.2,-0.1,0.));
#8530=CARTESIAN_POINT('Origin',(-6.4,-0.1,0.));
#8531=CARTESIAN_POINT('',(-6.4,0.0214285714285713,0.0809523809523809));
#8532=CARTESIAN_POINT('',(-5.56666666666667,0.2,0.2));
#8533=CARTESIAN_POINT('',(-5.78548644338118,0.15311004784689,0.168740031897927));
#8534=CARTESIAN_POINT('',(-6.4,-0.1,0.));
#8535=CARTESIAN_POINT('',(-6.4,-0.1,0.));
#8536=CARTESIAN_POINT('',(-2.2,-0.1,0.));
#8537=CARTESIAN_POINT('',(-5.225,0.2,0.2));
#8538=CARTESIAN_POINT('Origin',(-6.4,0.025,0.125));
#8539=CARTESIAN_POINT('',(-6.4,0.0214285714285713,0.2));
#8540=CARTESIAN_POINT('',(-6.4,0.0214285714285713,0.0625));
#8541=CARTESIAN_POINT('',(-6.4,-0.1,0.2));
#8542=CARTESIAN_POINT('',(-6.4,0.2875,0.2));
#8543=CARTESIAN_POINT('',(-6.4,-0.1,0.));
#8544=CARTESIAN_POINT('Origin',(-4.05,0.55,0.2));
#8545=CARTESIAN_POINT('',(-6.5,0.,0.2));
#8546=CARTESIAN_POINT('',(-6.5,0.,0.2));
#8547=CARTESIAN_POINT('',(-6.4,-0.1,0.2));
#8548=CARTESIAN_POINT('Origin',(-4.05,0.55,0.2));
#8549=CARTESIAN_POINT('',(-2.,0.133333333333333,0.2));
#8550=CARTESIAN_POINT('',(-1.6,0.6,0.2));
#8551=CARTESIAN_POINT('',(-2.,0.933333333333333,0.2));
#8552=CARTESIAN_POINT('',(-2.,0.875,0.2));
#8553=CARTESIAN_POINT('',(-2.5,0.6,0.2));
#8554=CARTESIAN_POINT('',(-2.5,0.6,0.2));
#8555=CARTESIAN_POINT('',(-5.1,0.3,0.2));
#8556=CARTESIAN_POINT('',(-5.1,0.3,0.2));
#8557=CARTESIAN_POINT('',(-6.5,0.,0.2));
#8558=CARTESIAN_POINT('Origin',(-1.6,1.2,0.));
#8559=CARTESIAN_POINT('',(-2.,0.933333333333333,0.));
#8560=CARTESIAN_POINT('',(-2.,0.933333333333333,0.));
#8561=CARTESIAN_POINT('',(-2.5,0.6,0.));
#8562=CARTESIAN_POINT('',(-2.5,0.6,0.));
#8563=CARTESIAN_POINT('',(-2.5,0.6,0.));
#8564=CARTESIAN_POINT('Origin',(-2.2,-0.1,0.));
#8565=CARTESIAN_POINT('',(-2.,0.133333333333333,0.));
#8566=CARTESIAN_POINT('',(-2.,0.133333333333334,0.));
#8567=CARTESIAN_POINT('',(-1.6,0.6,0.));
#8568=CARTESIAN_POINT('Origin',(-6.5,0.,0.));
#8569=CARTESIAN_POINT('',(-6.5,0.,0.));
#8570=CARTESIAN_POINT('',(-6.4,-0.1,0.));
#8571=CARTESIAN_POINT('',(-6.5,0.,0.));
#8572=CARTESIAN_POINT('Origin',(-5.1,0.3,0.));
#8573=CARTESIAN_POINT('',(-5.1,0.3,0.));
#8574=CARTESIAN_POINT('',(-5.1,0.3,0.));
#8575=CARTESIAN_POINT('',(-6.5,0.,0.));
#8576=CARTESIAN_POINT('Origin',(-2.5,0.6,0.));
#8577=CARTESIAN_POINT('',(-5.1,0.3,0.));
#8578=CARTESIAN_POINT('Origin',(0.,0.,0.));
#8579=CARTESIAN_POINT('',(-2.,1.2,0.));
#8580=CARTESIAN_POINT('',(-2.,0.,0.));
#8581=CARTESIAN_POINT('',(-1.2,1.2,0.));
#8582=CARTESIAN_POINT('',(-2.,1.2,0.));
#8583=CARTESIAN_POINT('',(-1.2,0.721110255092798,0.));
#8584=CARTESIAN_POINT('',(-1.2,1.2,0.));
#8585=CARTESIAN_POINT('',(0.993295878967653,0.986591757935306,0.));
#8586=CARTESIAN_POINT('Origin',(0.,0.,0.));
#8587=CARTESIAN_POINT('',(1.,1.,0.));
#8588=CARTESIAN_POINT('',(1.,1.,0.));
#8589=CARTESIAN_POINT('',(3.8,-1.9,0.));
#8590=CARTESIAN_POINT('',(3.8,-1.9,0.));
#8591=CARTESIAN_POINT('',(14.,-1.9,0.));
#8592=CARTESIAN_POINT('',(14.,-1.9,0.));
#8593=CARTESIAN_POINT('',(14.,-3.1,0.));
#8594=CARTESIAN_POINT('',(14.,-3.1,0.));
#8595=CARTESIAN_POINT('',(3.8,-3.1,0.));
#8596=CARTESIAN_POINT('',(3.8,-3.1,0.));
#8597=CARTESIAN_POINT('',(0.533017816115691,-1.29456247732709,0.));
#8598=CARTESIAN_POINT('',(0.,-1.,0.));
#8599=CARTESIAN_POINT('',(-1.4,0.,0.));
#8600=CARTESIAN_POINT('Origin',(0.,0.,0.));
#8601=CARTESIAN_POINT('',(-2.,0.,0.));
#8602=CARTESIAN_POINT('',(-1.2,0.,0.));
#8603=CARTESIAN_POINT('',(-2.,0.,0.));
#8604=CARTESIAN_POINT('Origin',(-2.,0.,0.));
#8605=CARTESIAN_POINT('',(-1.4,0.,0.6));
#8606=CARTESIAN_POINT('',(-1.4,0.,0.));
#8607=CARTESIAN_POINT('',(-2.,0.,0.6));
#8608=CARTESIAN_POINT('',(-1.2,0.,0.6));
#8609=CARTESIAN_POINT('',(-2.,0.,0.));
#8610=CARTESIAN_POINT('Origin',(-2.,1.2,0.));
#8611=CARTESIAN_POINT('',(-2.,1.2,0.6));
#8612=CARTESIAN_POINT('',(-2.,0.,0.6));
#8613=CARTESIAN_POINT('',(-2.,1.2,0.));
#8614=CARTESIAN_POINT('Origin',(-1.2,1.2,0.));
#8615=CARTESIAN_POINT('',(-1.2,1.2,0.6));
#8616=CARTESIAN_POINT('',(-2.,1.2,0.6));
#8617=CARTESIAN_POINT('',(-1.2,1.2,0.));
#8618=CARTESIAN_POINT('Origin',(-1.2,0.,0.));
#8619=CARTESIAN_POINT('',(-1.2,0.721110255092798,0.6));
#8620=CARTESIAN_POINT('',(-1.2,0.721110255092798,0.));
#8621=CARTESIAN_POINT('',(-1.2,1.2,0.6));
#8622=CARTESIAN_POINT('Origin',(0.,0.,0.));
#8623=CARTESIAN_POINT('',(0.533017816115691,-1.29456247732709,0.6));
#8624=CARTESIAN_POINT('',(0.533017816115691,-1.29456247732709,0.));
#8625=CARTESIAN_POINT('Origin',(0.,0.,0.6));
#8626=CARTESIAN_POINT('Origin',(0.,0.,0.));
#8627=CARTESIAN_POINT('',(0.993295878967653,0.986591757935306,0.6));
#8628=CARTESIAN_POINT('Origin',(0.,0.,0.6));
#8629=CARTESIAN_POINT('',(0.993295878967653,0.986591757935306,0.));
#8630=CARTESIAN_POINT('Origin',(0.,0.,0.6));
#8631=CARTESIAN_POINT('',(3.8,-3.1,0.6));
#8632=CARTESIAN_POINT('',(0.,-1.,0.6));
#8633=CARTESIAN_POINT('',(14.,-3.1,0.6));
#8634=CARTESIAN_POINT('',(3.8,-3.1,0.6));
#8635=CARTESIAN_POINT('',(14.,-1.9,0.6));
#8636=CARTESIAN_POINT('',(14.,-3.1,0.6));
#8637=CARTESIAN_POINT('',(3.8,-1.9,0.6));
#8638=CARTESIAN_POINT('',(14.,-1.9,0.6));
#8639=CARTESIAN_POINT('',(1.,1.,0.6));
#8640=CARTESIAN_POINT('',(3.8,-1.9,0.6));
#8641=CARTESIAN_POINT('',(1.,1.,0.6));
#8642=CARTESIAN_POINT('Origin',(0.,-1.,0.));
#8643=CARTESIAN_POINT('',(3.8,-3.1,0.));
#8644=CARTESIAN_POINT('Origin',(1.,1.,0.));
#8645=CARTESIAN_POINT('',(1.,1.,0.));
#8646=CARTESIAN_POINT('Origin',(3.8,-1.9,0.));
#8647=CARTESIAN_POINT('',(3.8,-1.9,0.));
#8648=CARTESIAN_POINT('Origin',(14.,-1.9,0.));
#8649=CARTESIAN_POINT('',(14.,-1.9,0.));
#8650=CARTESIAN_POINT('Origin',(14.,-3.1,0.));
#8651=CARTESIAN_POINT('',(14.,-3.1,0.));
#8652=CARTESIAN_POINT('Origin',(3.8,-3.1,0.));
#18558=UNCERTAINTY_MEASURE_WITH_UNIT(LENGTH_MEASURE(0.001),#18581,
'DISTANCE_ACCURACY_VALUE',
'Maximum model space distance between geometric entities at asserted c
onnectivities');
#18568=UNCERTAINTY_MEASURE_WITH_UNIT(LENGTH_MEASURE(0.001),#18581,
'DISTANCE_ACCURACY_VALUE',
'Maximum model space distance between geometric entities at asserted c
onnectivities');
#18570=(
GEOMETRIC_REPRESENTATION_CONTEXT(3)
GLOBAL_UNCERTAINTY_ASSIGNED_CONTEXT((#18558))
GLOBAL_UNIT_ASSIGNED_CONTEXT((#18581,#18583,#18584))
REPRESENTATION_CONTEXT('','3D')
);
#18580=(
GEOMETRIC_REPRESENTATION_CONTEXT(3)
GLOBAL_UNCERTAINTY_ASSIGNED_CONTEXT((#18568))
GLOBAL_UNIT_ASSIGNED_CONTEXT((#18581,#18583,#18584))
REPRESENTATION_CONTEXT('','3D')
);
#18581=(
LENGTH_UNIT()
NAMED_UNIT(*)
SI_UNIT(.CENTI.,.METRE.)
);
#18583=(
NAMED_UNIT(*)
PLANE_ANGLE_UNIT()
SI_UNIT($,.RADIAN.)
);
#18584=(
NAMED_UNIT(*)
SI_UNIT($,.STERADIAN.)
SOLID_ANGLE_UNIT()
);
#18586=SHAPE_DEFINITION_REPRESENTATION(#18597,#18624);
#18597=PRODUCT_DEFINITION_SHAPE('',$,#18636);
#18624=SHAPE_REPRESENTATION('',(#6654),#18570);
#18634=PRODUCT_DEFINITION_CONTEXT('part definition',#18669,'design');
#18636=PRODUCT_DEFINITION('Forged jaw and handle',
'Forged jaw and handle',#18647,#18634);
#18647=PRODUCT_DEFINITION_FORMATION('',$,#18672);
#18669=APPLICATION_CONTEXT(
'Core Data for Automotive Mechanical Design Process');
#18670=PRODUCT_CONTEXT('part definition',#18669,'mechanical');
#18672=PRODUCT('Forged jaw and handle','Forged jaw and handle',$,(#18670));
#18683=PRESENTATION_STYLE_ASSIGNMENT((#18691));
#18691=SURFACE_STYLE_USAGE(.BOTH.,#18699);
#18699=SURFACE_SIDE_STYLE('',(#18707));
#18707=SURFACE_STYLE_FILL_AREA(#18715);
#18715=FILL_AREA_STYLE('Tool steel gray',(#18723));
#18723=FILL_AREA_STYLE_COLOUR('Tool steel gray',#18731);
#18731=COLOUR_RGB('Tool steel gray',0.607843137254902,0.643137254901961,
0.698039215686274);
ENDSEC;
END-ISO-10303-21;
